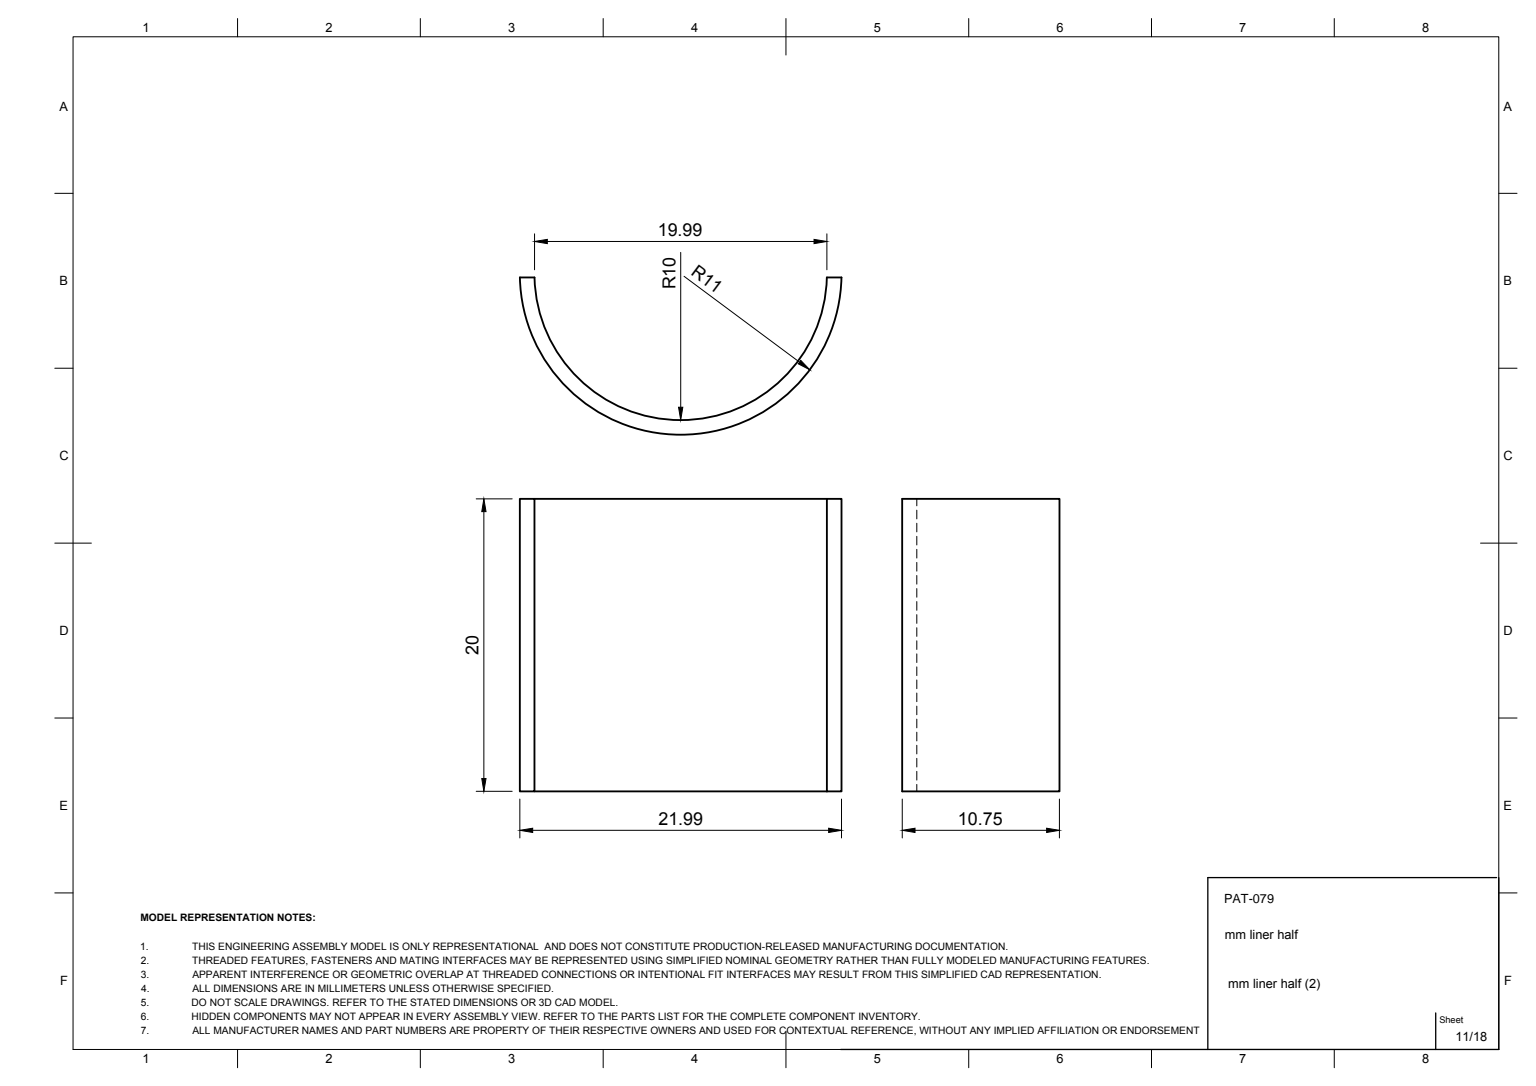
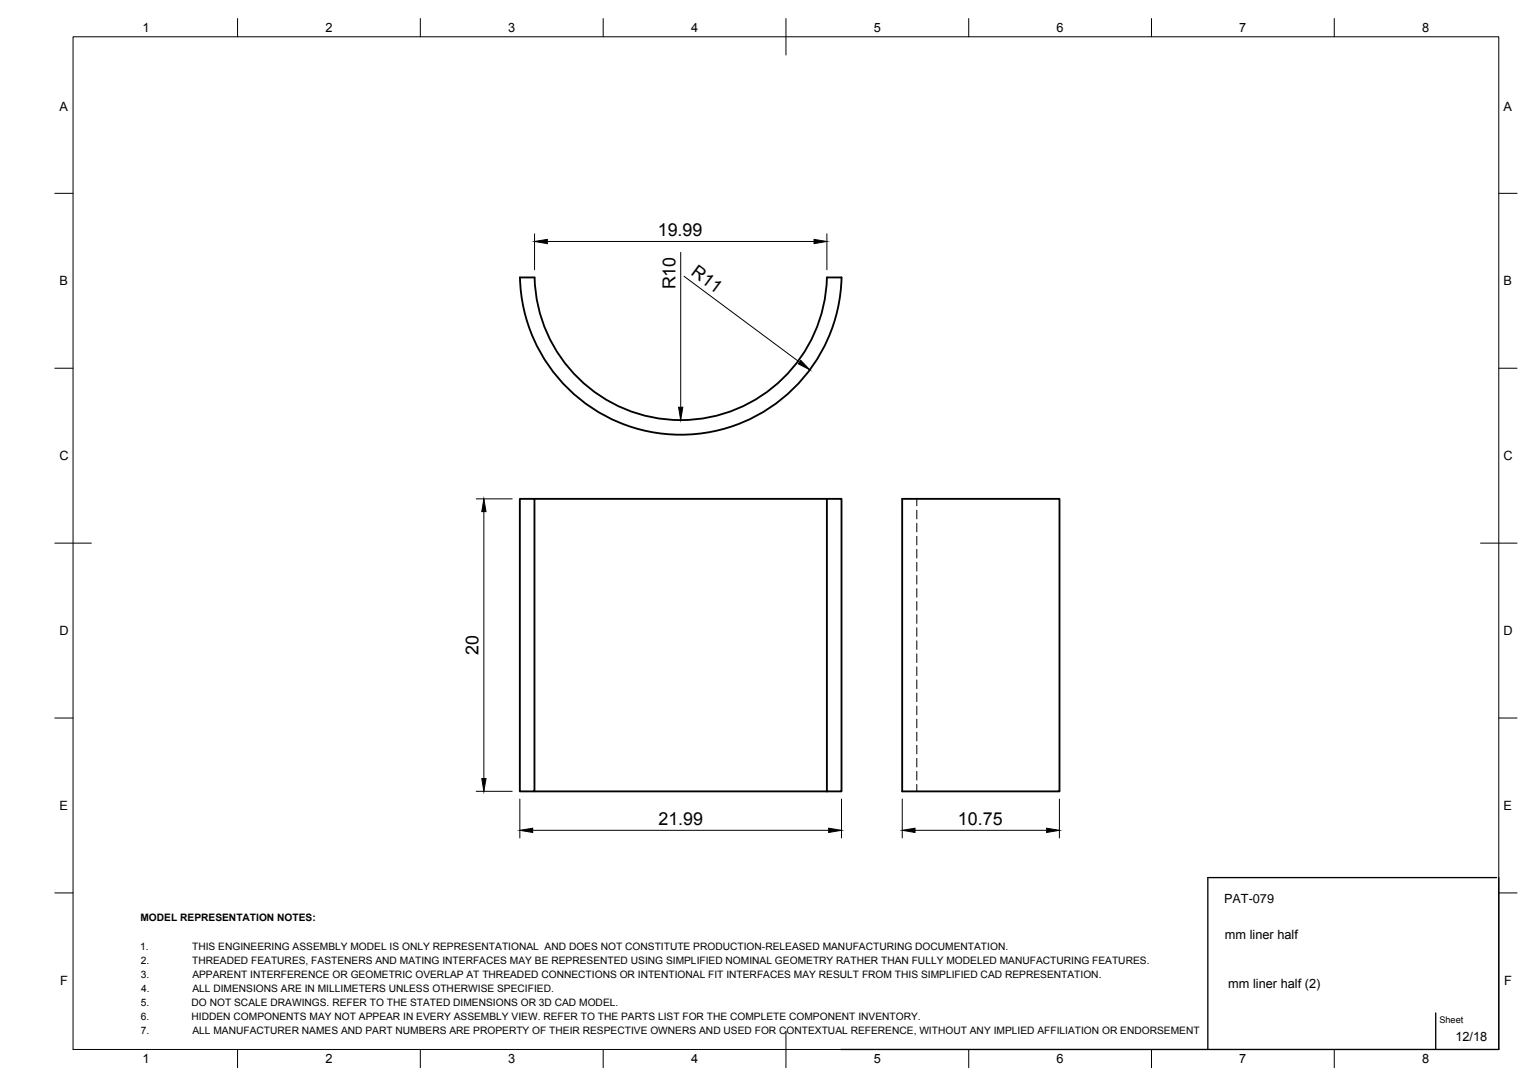
ISO-10303-21;
HEADER;
/* Generated by software containing ST-Developer
 * from STEP Tools, Inc. (www.steptools.com) 
 */

FILE_DESCRIPTION(
/* description */ ('Pipe clamp stand with threaded column'),
/* implementation_level */ '2;1');

FILE_NAME(
/* name */ 'mm liner half.step',
/* time_stamp */ '2026-10-27T10:55:48-07:00',
/* author */ (''),
/* organization */ (''),
/* preprocessor_version */ 'ST-DEVELOPER v20.2',
/* originating_system */ 'Autodesk Translation Framework v15.17.0.0',
/* authorisation */ '');

FILE_SCHEMA (('AUTOMOTIVE_DESIGN { 1 0 10303 214 3 1 1 }'));
ENDSEC;

DATA;
#10=MECHANICAL_DESIGN_GEOMETRIC_PRESENTATION_REPRESENTATION('',(#751),#34433);
#703=SHAPE_REPRESENTATION_RELATIONSHIP('SRR','None',#34545,#725);
#725=ADVANCED_BREP_SHAPE_REPRESENTATION('',(#781),#34413);
#751=STYLED_ITEM('',(#34736),#781);
#781=MANIFOLD_SOLID_BREP('Body1',#8778);
#911=PLANE('',#9378);
#912=PLANE('',#9379);
#913=PLANE('',#9380);
#914=PLANE('',#9387);
#1316=FACE_OUTER_BOUND('',#1836,.T.);
#1317=FACE_OUTER_BOUND('',#1837,.T.);
#1318=FACE_OUTER_BOUND('',#1838,.T.);
#1319=FACE_OUTER_BOUND('',#1839,.T.);
#1320=FACE_OUTER_BOUND('',#1840,.T.);
#1321=FACE_OUTER_BOUND('',#1841,.T.);
#1836=EDGE_LOOP('',(#7007,#7008,#7009,#7010));
#1837=EDGE_LOOP('',(#7011,#7012,#7013,#7014));
#1838=EDGE_LOOP('',(#7015,#7016,#7017,#7018));
#1839=EDGE_LOOP('',(#7019,#7020,#7021,#7022));
#1840=EDGE_LOOP('',(#7023,#7024,#7025,#7026));
#1841=EDGE_LOOP('',(#7027,#7028,#7029,#7030));
#2383=LINE('',#28278,#3000);
#2384=LINE('',#28280,#3001);
#2385=LINE('',#28282,#3002);
#2386=LINE('',#28283,#3003);
#2387=LINE('',#28287,#3004);
#2388=LINE('',#28289,#3005);
#2389=LINE('',#28291,#3006);
#2390=LINE('',#28292,#3007);
#3000=VECTOR('',#10704,1.);
#3001=VECTOR('',#10705,1.);
#3002=VECTOR('',#10706,1.);
#3003=VECTOR('',#10707,1.);
#3004=VECTOR('',#10710,1.);
#3005=VECTOR('',#10711,1.);
#3006=VECTOR('',#10712,1.);
#3007=VECTOR('',#10713,1.);
#3366=CIRCLE('',#9381,1.1);
#3367=CIRCLE('',#9382,1.);
#3368=CIRCLE('',#9384,1.);
#3369=CIRCLE('',#9386,1.1);
#3942=VERTEX_POINT('',#28276);
#3943=VERTEX_POINT('',#28277);
#3944=VERTEX_POINT('',#28279);
#3945=VERTEX_POINT('',#28281);
#3946=VERTEX_POINT('',#28285);
#3947=VERTEX_POINT('',#28286);
#3948=VERTEX_POINT('',#28288);
#3949=VERTEX_POINT('',#28290);
#5017=EDGE_CURVE('',#3942,#3943,#2383,.T.);
#5018=EDGE_CURVE('',#3944,#3942,#2384,.T.);
#5019=EDGE_CURVE('',#3945,#3944,#2385,.T.);
#5020=EDGE_CURVE('',#3943,#3945,#2386,.T.);
#5021=EDGE_CURVE('',#3946,#3947,#2387,.T.);
#5022=EDGE_CURVE('',#3948,#3946,#2388,.T.);
#5023=EDGE_CURVE('',#3949,#3948,#2389,.T.);
#5024=EDGE_CURVE('',#3947,#3949,#2390,.T.);
#5025=EDGE_CURVE('',#3943,#3946,#3366,.T.);
#5026=EDGE_CURVE('',#3948,#3945,#3367,.T.);
#5027=EDGE_CURVE('',#3949,#3944,#3368,.T.);
#5028=EDGE_CURVE('',#3942,#3947,#3369,.T.);
#7007=ORIENTED_EDGE('',*,*,#5017,.F.);
#7008=ORIENTED_EDGE('',*,*,#5018,.F.);
#7009=ORIENTED_EDGE('',*,*,#5019,.F.);
#7010=ORIENTED_EDGE('',*,*,#5020,.F.);
#7011=ORIENTED_EDGE('',*,*,#5021,.F.);
#7012=ORIENTED_EDGE('',*,*,#5022,.F.);
#7013=ORIENTED_EDGE('',*,*,#5023,.F.);
#7014=ORIENTED_EDGE('',*,*,#5024,.F.);
#7015=ORIENTED_EDGE('',*,*,#5022,.T.);
#7016=ORIENTED_EDGE('',*,*,#5025,.F.);
#7017=ORIENTED_EDGE('',*,*,#5020,.T.);
#7018=ORIENTED_EDGE('',*,*,#5026,.F.);
#7019=ORIENTED_EDGE('',*,*,#5023,.T.);
#7020=ORIENTED_EDGE('',*,*,#5026,.T.);
#7021=ORIENTED_EDGE('',*,*,#5019,.T.);
#7022=ORIENTED_EDGE('',*,*,#5027,.F.);
#7023=ORIENTED_EDGE('',*,*,#5021,.T.);
#7024=ORIENTED_EDGE('',*,*,#5028,.F.);
#7025=ORIENTED_EDGE('',*,*,#5017,.T.);
#7026=ORIENTED_EDGE('',*,*,#5025,.T.);
#7027=ORIENTED_EDGE('',*,*,#5024,.T.);
#7028=ORIENTED_EDGE('',*,*,#5027,.T.);
#7029=ORIENTED_EDGE('',*,*,#5018,.T.);
#7030=ORIENTED_EDGE('',*,*,#5028,.T.);
#8215=CYLINDRICAL_SURFACE('',#9383,1.);
#8216=CYLINDRICAL_SURFACE('',#9385,1.1);
#8553=ADVANCED_FACE('',(#1316),#911,.F.);
#8554=ADVANCED_FACE('',(#1317),#912,.F.);
#8555=ADVANCED_FACE('',(#1318),#913,.F.);
#8556=ADVANCED_FACE('',(#1319),#8215,.F.);
#8557=ADVANCED_FACE('',(#1320),#8216,.T.);
#8558=ADVANCED_FACE('',(#1321),#914,.T.);
#8778=CLOSED_SHELL('',(#8553,#8554,#8555,#8556,#8557,#8558));
#9377=AXIS2_PLACEMENT_3D('',#28274,#10700,#10701);
#9378=AXIS2_PLACEMENT_3D('',#28275,#10702,#10703);
#9379=AXIS2_PLACEMENT_3D('',#28284,#10708,#10709);
#9380=AXIS2_PLACEMENT_3D('',#28293,#10714,#10715);
#9381=AXIS2_PLACEMENT_3D('',#28294,#10716,#10717);
#9382=AXIS2_PLACEMENT_3D('',#28295,#10718,#10719);
#9383=AXIS2_PLACEMENT_3D('',#28296,#10720,#10721);
#9384=AXIS2_PLACEMENT_3D('',#28297,#10722,#10723);
#9385=AXIS2_PLACEMENT_3D('',#28298,#10724,#10725);
#9386=AXIS2_PLACEMENT_3D('',#28299,#10726,#10727);
#9387=AXIS2_PLACEMENT_3D('',#28300,#10728,#10729);
#10700=DIRECTION('axis',(0.,0.,1.));
#10701=DIRECTION('refdir',(1.,0.,0.));
#10702=DIRECTION('center_axis',(0.,0.,-1.));
#10703=DIRECTION('ref_axis',(-1.,0.,0.));
#10704=DIRECTION('',(0.,-1.,0.));
#10705=DIRECTION('',(1.,0.,0.));
#10706=DIRECTION('',(0.,1.,0.));
#10707=DIRECTION('',(-1.,0.,0.));
#10708=DIRECTION('center_axis',(0.,0.,-1.));
#10709=DIRECTION('ref_axis',(-1.,0.,0.));
#10710=DIRECTION('',(0.,1.,0.));
#10711=DIRECTION('',(-1.,0.,0.));
#10712=DIRECTION('',(0.,-1.,0.));
#10713=DIRECTION('',(1.,0.,0.));
#10714=DIRECTION('center_axis',(0.,1.,0.));
#10715=DIRECTION('ref_axis',(1.,0.,0.));
#10716=DIRECTION('center_axis',(0.,1.,0.));
#10717=DIRECTION('ref_axis',(1.,0.,0.));
#10718=DIRECTION('center_axis',(0.,-1.,0.));
#10719=DIRECTION('ref_axis',(1.,0.,0.));
#10720=DIRECTION('center_axis',(0.,1.,0.));
#10721=DIRECTION('ref_axis',(1.,0.,0.));
#10722=DIRECTION('center_axis',(0.,-1.,0.));
#10723=DIRECTION('ref_axis',(1.,0.,0.));
#10724=DIRECTION('center_axis',(0.,1.,0.));
#10725=DIRECTION('ref_axis',(1.,0.,0.));
#10726=DIRECTION('center_axis',(0.,1.,0.));
#10727=DIRECTION('ref_axis',(1.,0.,0.));
#10728=DIRECTION('center_axis',(0.,1.,0.));
#10729=DIRECTION('ref_axis',(1.,0.,0.));
#28274=CARTESIAN_POINT('',(0.,0.,0.));
#28275=CARTESIAN_POINT('Origin',(4.,-1.1,17.975));
#28276=CARTESIAN_POINT('',(1.09971587239614,1.,17.975));
#28277=CARTESIAN_POINT('',(1.09971587239614,-1.,17.975));
#28278=CARTESIAN_POINT('',(1.09971587239614,-1.,17.975));
#28279=CARTESIAN_POINT('',(0.99968745115661,1.,17.975));
#28280=CARTESIAN_POINT('',(2.,1.,17.975));
#28281=CARTESIAN_POINT('',(0.99968745115661,-1.,17.975));
#28282=CARTESIAN_POINT('',(0.99968745115661,-1.,17.975));
#28283=CARTESIAN_POINT('',(2.,-1.,17.975));
#28284=CARTESIAN_POINT('Origin',(4.,-1.1,17.975));
#28285=CARTESIAN_POINT('',(-1.09971587239614,-1.,17.975));
#28286=CARTESIAN_POINT('',(-1.09971587239614,1.,17.975));
#28287=CARTESIAN_POINT('',(-1.09971587239614,-1.,17.975));
#28288=CARTESIAN_POINT('',(-0.99968745115661,-1.,17.975));
#28289=CARTESIAN_POINT('',(2.,-1.,17.975));
#28290=CARTESIAN_POINT('',(-0.99968745115661,1.,17.975));
#28291=CARTESIAN_POINT('',(-0.99968745115661,-1.,17.975));
#28292=CARTESIAN_POINT('',(2.,1.,17.975));
#28293=CARTESIAN_POINT('Origin',(0.,-1.,18.));
#28294=CARTESIAN_POINT('Origin',(0.,-1.,18.));
#28295=CARTESIAN_POINT('Origin',(0.,-1.,18.));
#28296=CARTESIAN_POINT('Origin',(0.,-1.,18.));
#28297=CARTESIAN_POINT('Origin',(0.,1.,18.));
#28298=CARTESIAN_POINT('Origin',(0.,-1.,18.));
#28299=CARTESIAN_POINT('Origin',(0.,1.,18.));
#28300=CARTESIAN_POINT('Origin',(0.,1.,18.));
#34384=UNCERTAINTY_MEASURE_WITH_UNIT(LENGTH_MEASURE(0.001),#34434,
'DISTANCE_ACCURACY_VALUE',
'Maximum model space distance between geometric entities at asserted c
onnectivities');
#34404=UNCERTAINTY_MEASURE_WITH_UNIT(LENGTH_MEASURE(0.001),#34434,
'DISTANCE_ACCURACY_VALUE',
'Maximum model space distance between geometric entities at asserted c
onnectivities');
#34413=(
GEOMETRIC_REPRESENTATION_CONTEXT(3)
GLOBAL_UNCERTAINTY_ASSIGNED_CONTEXT((#34384))
GLOBAL_UNIT_ASSIGNED_CONTEXT((#34434,#34436,#34437))
REPRESENTATION_CONTEXT('','3D')
);
#34433=(
GEOMETRIC_REPRESENTATION_CONTEXT(3)
GLOBAL_UNCERTAINTY_ASSIGNED_CONTEXT((#34404))
GLOBAL_UNIT_ASSIGNED_CONTEXT((#34434,#34436,#34437))
REPRESENTATION_CONTEXT('','3D')
);
#34434=(
LENGTH_UNIT()
NAMED_UNIT(*)
SI_UNIT(.CENTI.,.METRE.)
);
#34436=(
NAMED_UNIT(*)
PLANE_ANGLE_UNIT()
SI_UNIT($,.RADIAN.)
);
#34437=(
NAMED_UNIT(*)
SI_UNIT($,.STERADIAN.)
SOLID_ANGLE_UNIT()
);
#34446=SHAPE_DEFINITION_REPRESENTATION(#34474,#34545);
#34474=PRODUCT_DEFINITION_SHAPE('',$,#34574);
#34545=SHAPE_REPRESENTATION('',(#9377),#34413);
#34565=PRODUCT_DEFINITION_CONTEXT('part definition',#34651,'design');
#34574=PRODUCT_DEFINITION('mm liner half','mm liner half',#34602,#34565);
#34602=PRODUCT_DEFINITION_FORMATION('',$,#34661);
#34651=APPLICATION_CONTEXT(
'Core Data for Automotive Mechanical Design Process');
#34652=PRODUCT_CONTEXT('part definition',#34651,'mechanical');
#34661=PRODUCT('mm liner half','mm liner half','mm liner half',(#34652));
#34730=COLOUR_RGB('Sky Blue',0.24,0.69,0.87);
#34731=FILL_AREA_STYLE_COLOUR('',#34730);
#34732=FILL_AREA_STYLE('',(#34731));
#34733=SURFACE_STYLE_FILL_AREA(#34732);
#34734=SURFACE_SIDE_STYLE('',(#34733));
#34735=SURFACE_STYLE_USAGE(.BOTH.,#34734);
#34736=PRESENTATION_STYLE_ASSIGNMENT((#34735));
ENDSEC;
END-ISO-10303-21;
